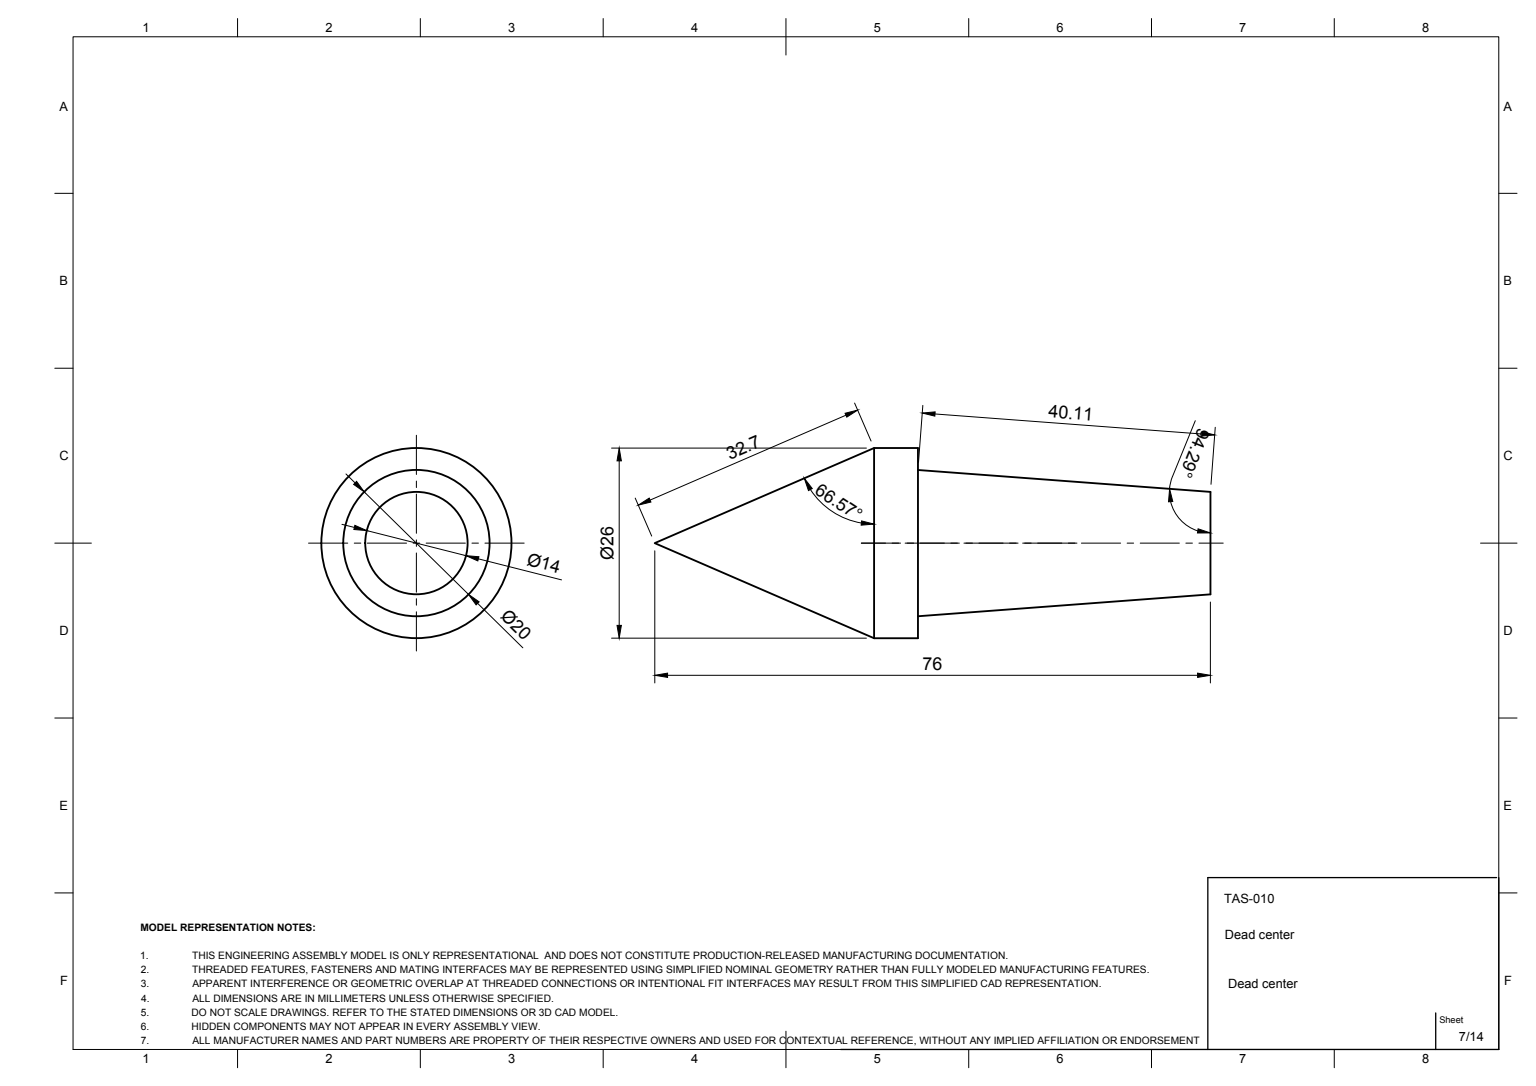
ISO-10303-21;
HEADER;
/* Generated by software containing ST-Developer
 * from STEP Tools, Inc. (www.steptools.com) 
 */

FILE_DESCRIPTION(
/* description */ (
'Independent keyed-quill tailstock, native coupled50mm slider andM16x2
 feed screw, conical dead center, bronze sleeves/thrust washers, cross
-pinned handwheel and bolted guide key. Custom center taper; no standa
rd taper compatibility, machine-bed compatibility or load rating assig
ned.'),
/* implementation_level */ '2;1');

FILE_NAME(
/* name */ 'Dead center.step',
/* time_stamp */ '2026-11-14T07:17:36-08:00',
/* author */ (''),
/* organization */ (''),
/* preprocessor_version */ 'ST-DEVELOPER v20.2',
/* originating_system */ 'Autodesk Translation Framework v15.17.0.0',
/* authorisation */ '');

FILE_SCHEMA (('AUTOMOTIVE_DESIGN { 1 0 10303 214 3 1 1 }'));
ENDSEC;

DATA;
#10=MECHANICAL_DESIGN_GEOMETRIC_PRESENTATION_REPRESENTATION('',(#157),#289387);
#112=CONICAL_SURFACE('',#17528,8.5,0.0748598477107669);
#113=CONICAL_SURFACE('',#17534,13.,0.408907828950925);
#123=SHAPE_REPRESENTATION_RELATIONSHIP('SRR','None',#289458,#140);
#140=ADVANCED_BREP_SHAPE_REPRESENTATION('',(#174),#289374);
#157=STYLED_ITEM('',(#289548),#174);
#174=MANIFOLD_SOLID_BREP('Body1',#16845);
#222=FACE_BOUND('',#1521,.T.);
#352=PLANE('',#17526);
#353=PLANE('',#17530);
#833=FACE_OUTER_BOUND('',#1518,.T.);
#834=FACE_OUTER_BOUND('',#1519,.T.);
#835=FACE_OUTER_BOUND('',#1520,.T.);
#836=FACE_OUTER_BOUND('',#1522,.T.);
#837=FACE_OUTER_BOUND('',#1523,.T.);
#1518=EDGE_LOOP('',(#13659));
#1519=EDGE_LOOP('',(#13660,#13661,#13662,#13663));
#1520=EDGE_LOOP('',(#13664));
#1521=EDGE_LOOP('',(#13665));
#1522=EDGE_LOOP('',(#13666,#13667,#13668,#13669));
#1523=EDGE_LOOP('',(#13670,#13671,#13672));
#1895=CIRCLE('',#17527,7.);
#1896=CIRCLE('',#17529,10.);
#1897=CIRCLE('',#17531,13.);
#1898=CIRCLE('',#17533,13.);
#4326=LINE('',#185153,#4963);
#4327=LINE('',#185160,#4964);
#4328=LINE('',#185163,#4965);
#4963=VECTOR('',#19242,8.5);
#4964=VECTOR('',#19251,13.);
#4965=VECTOR('',#19254,13.);
#6575=VERTEX_POINT('',#185148);
#6576=VERTEX_POINT('',#185151);
#6577=VERTEX_POINT('',#185155);
#6578=VERTEX_POINT('',#185158);
#6579=VERTEX_POINT('',#185162);
#9141=EDGE_CURVE('',#6575,#6575,#1895,.T.);
#9142=EDGE_CURVE('',#6576,#6576,#1896,.T.);
#9143=EDGE_CURVE('',#6576,#6575,#4326,.T.);
#9144=EDGE_CURVE('',#6577,#6577,#1897,.T.);
#9145=EDGE_CURVE('',#6578,#6578,#1898,.T.);
#9146=EDGE_CURVE('',#6578,#6577,#4327,.T.);
#9147=EDGE_CURVE('',#6578,#6579,#4328,.T.);
#13659=ORIENTED_EDGE('',*,*,#9141,.F.);
#13660=ORIENTED_EDGE('',*,*,#9142,.F.);
#13661=ORIENTED_EDGE('',*,*,#9143,.T.);
#13662=ORIENTED_EDGE('',*,*,#9141,.T.);
#13663=ORIENTED_EDGE('',*,*,#9143,.F.);
#13664=ORIENTED_EDGE('',*,*,#9144,.F.);
#13665=ORIENTED_EDGE('',*,*,#9142,.T.);
#13666=ORIENTED_EDGE('',*,*,#9145,.F.);
#13667=ORIENTED_EDGE('',*,*,#9146,.T.);
#13668=ORIENTED_EDGE('',*,*,#9144,.T.);
#13669=ORIENTED_EDGE('',*,*,#9146,.F.);
#13670=ORIENTED_EDGE('',*,*,#9145,.T.);
#13671=ORIENTED_EDGE('',*,*,#9147,.T.);
#13672=ORIENTED_EDGE('',*,*,#9147,.F.);
#16037=CYLINDRICAL_SURFACE('',#17532,13.);
#16601=ADVANCED_FACE('',(#833),#352,.T.);
#16602=ADVANCED_FACE('',(#834),#112,.T.);
#16603=ADVANCED_FACE('',(#835,#222),#353,.T.);
#16604=ADVANCED_FACE('',(#836),#16037,.T.);
#16605=ADVANCED_FACE('',(#837),#113,.T.);
#16845=CLOSED_SHELL('',(#16601,#16602,#16603,#16604,#16605));
#17525=AXIS2_PLACEMENT_3D('',#185146,#19232,#19233);
#17526=AXIS2_PLACEMENT_3D('',#185147,#19234,#19235);
#17527=AXIS2_PLACEMENT_3D('',#185149,#19236,#19237);
#17528=AXIS2_PLACEMENT_3D('',#185150,#19238,#19239);
#17529=AXIS2_PLACEMENT_3D('',#185152,#19240,#19241);
#17530=AXIS2_PLACEMENT_3D('',#185154,#19243,#19244);
#17531=AXIS2_PLACEMENT_3D('',#185156,#19245,#19246);
#17532=AXIS2_PLACEMENT_3D('',#185157,#19247,#19248);
#17533=AXIS2_PLACEMENT_3D('',#185159,#19249,#19250);
#17534=AXIS2_PLACEMENT_3D('',#185161,#19252,#19253);
#19232=DIRECTION('axis',(0.,0.,1.));
#19233=DIRECTION('refdir',(1.,0.,0.));
#19234=DIRECTION('center_axis',(0.,0.,-1.));
#19235=DIRECTION('ref_axis',(-1.,0.,0.));
#19236=DIRECTION('center_axis',(0.,0.,1.));
#19237=DIRECTION('ref_axis',(1.,0.,0.));
#19238=DIRECTION('center_axis',(0.,0.,1.));
#19239=DIRECTION('ref_axis',(1.,0.,0.));
#19240=DIRECTION('center_axis',(0.,0.,1.));
#19241=DIRECTION('ref_axis',(1.,0.,0.));
#19242=DIRECTION('',(0.0747899482416343,9.15912707225136E-18,-0.997199309888457));
#19243=DIRECTION('center_axis',(0.,0.,-1.));
#19244=DIRECTION('ref_axis',(-1.,0.,0.));
#19245=DIRECTION('center_axis',(0.,0.,1.));
#19246=DIRECTION('ref_axis',(1.,0.,0.));
#19247=DIRECTION('center_axis',(0.,0.,1.));
#19248=DIRECTION('ref_axis',(1.,0.,0.));
#19249=DIRECTION('center_axis',(0.,0.,1.));
#19250=DIRECTION('ref_axis',(1.,0.,0.));
#19251=DIRECTION('',(0.,0.,-1.));
#19252=DIRECTION('center_axis',(0.,0.,-1.));
#19253=DIRECTION('ref_axis',(1.,0.,0.));
#19254=DIRECTION('',(0.3976074376343,-4.86928675816027E-17,0.917555625309924));
#185146=CARTESIAN_POINT('',(0.,0.,0.));
#185147=CARTESIAN_POINT('Origin',(7.,0.,120.));
#185148=CARTESIAN_POINT('',(-7.,-8.57252759403147E-16,120.));
#185149=CARTESIAN_POINT('Origin',(0.,0.,120.));
#185150=CARTESIAN_POINT('Origin',(0.,0.,140.));
#185151=CARTESIAN_POINT('',(-10.,-1.22464679914735E-15,160.));
#185152=CARTESIAN_POINT('Origin',(0.,0.,160.));
#185153=CARTESIAN_POINT('',(-8.5,-1.04094977927525E-15,140.));
#185154=CARTESIAN_POINT('Origin',(13.,0.,160.));
#185155=CARTESIAN_POINT('',(-13.,-1.59204083889156E-15,160.));
#185156=CARTESIAN_POINT('Origin',(0.,0.,160.));
#185157=CARTESIAN_POINT('Origin',(0.,0.,163.));
#185158=CARTESIAN_POINT('',(-13.,-1.59204083889156E-15,166.));
#185159=CARTESIAN_POINT('Origin',(0.,0.,166.));
#185160=CARTESIAN_POINT('',(-13.,-1.59204083889156E-15,163.));
#185161=CARTESIAN_POINT('Origin',(0.,0.,166.));
#185162=CARTESIAN_POINT('',(0.,0.,196.));
#185163=CARTESIAN_POINT('',(-13.,1.59204083889156E-15,166.));
#289355=UNCERTAINTY_MEASURE_WITH_UNIT(LENGTH_MEASURE(0.01),#289388,
'DISTANCE_ACCURACY_VALUE',
'Maximum model space distance between geometric entities at asserted c
onnectivities');
#289368=UNCERTAINTY_MEASURE_WITH_UNIT(LENGTH_MEASURE(0.01),#289388,
'DISTANCE_ACCURACY_VALUE',
'Maximum model space distance between geometric entities at asserted c
onnectivities');
#289374=(
GEOMETRIC_REPRESENTATION_CONTEXT(3)
GLOBAL_UNCERTAINTY_ASSIGNED_CONTEXT((#289355))
GLOBAL_UNIT_ASSIGNED_CONTEXT((#289388,#289390,#289391))
REPRESENTATION_CONTEXT('','3D')
);
#289387=(
GEOMETRIC_REPRESENTATION_CONTEXT(3)
GLOBAL_UNCERTAINTY_ASSIGNED_CONTEXT((#289368))
GLOBAL_UNIT_ASSIGNED_CONTEXT((#289388,#289390,#289391))
REPRESENTATION_CONTEXT('','3D')
);
#289388=(
LENGTH_UNIT()
NAMED_UNIT(*)
SI_UNIT(.MILLI.,.METRE.)
);
#289390=(
NAMED_UNIT(*)
PLANE_ANGLE_UNIT()
SI_UNIT($,.RADIAN.)
);
#289391=(
NAMED_UNIT(*)
SI_UNIT($,.STERADIAN.)
SOLID_ANGLE_UNIT()
);
#289397=SHAPE_DEFINITION_REPRESENTATION(#289415,#289458);
#289415=PRODUCT_DEFINITION_SHAPE('',$,#289477);
#289458=SHAPE_REPRESENTATION('',(#17525),#289374);
#289471=PRODUCT_DEFINITION_CONTEXT('part definition',#289527,'design');
#289477=PRODUCT_DEFINITION('Dead center','Dead center',#289495,#289471);
#289495=PRODUCT_DEFINITION_FORMATION('',$,#289534);
#289527=APPLICATION_CONTEXT(
'Core Data for Automotive Mechanical Design Process');
#289528=PRODUCT_CONTEXT('part definition',#289527,'mechanical');
#289534=PRODUCT('Dead center','Dead center',$,(#289528));
#289548=PRESENTATION_STYLE_ASSIGNMENT((#289555));
#289555=SURFACE_STYLE_USAGE(.BOTH.,#289562);
#289562=SURFACE_SIDE_STYLE('',(#289569));
#289569=SURFACE_STYLE_FILL_AREA(#289576);
#289576=FILL_AREA_STYLE('Opaque(104,114,127)',(#289583));
#289583=FILL_AREA_STYLE_COLOUR('Opaque(104,114,127)',#289590);
#289590=COLOUR_RGB('Opaque(104,114,127)',0.407843137254902,0.447058823529412,
0.498039215686275);
ENDSEC;
END-ISO-10303-21;
